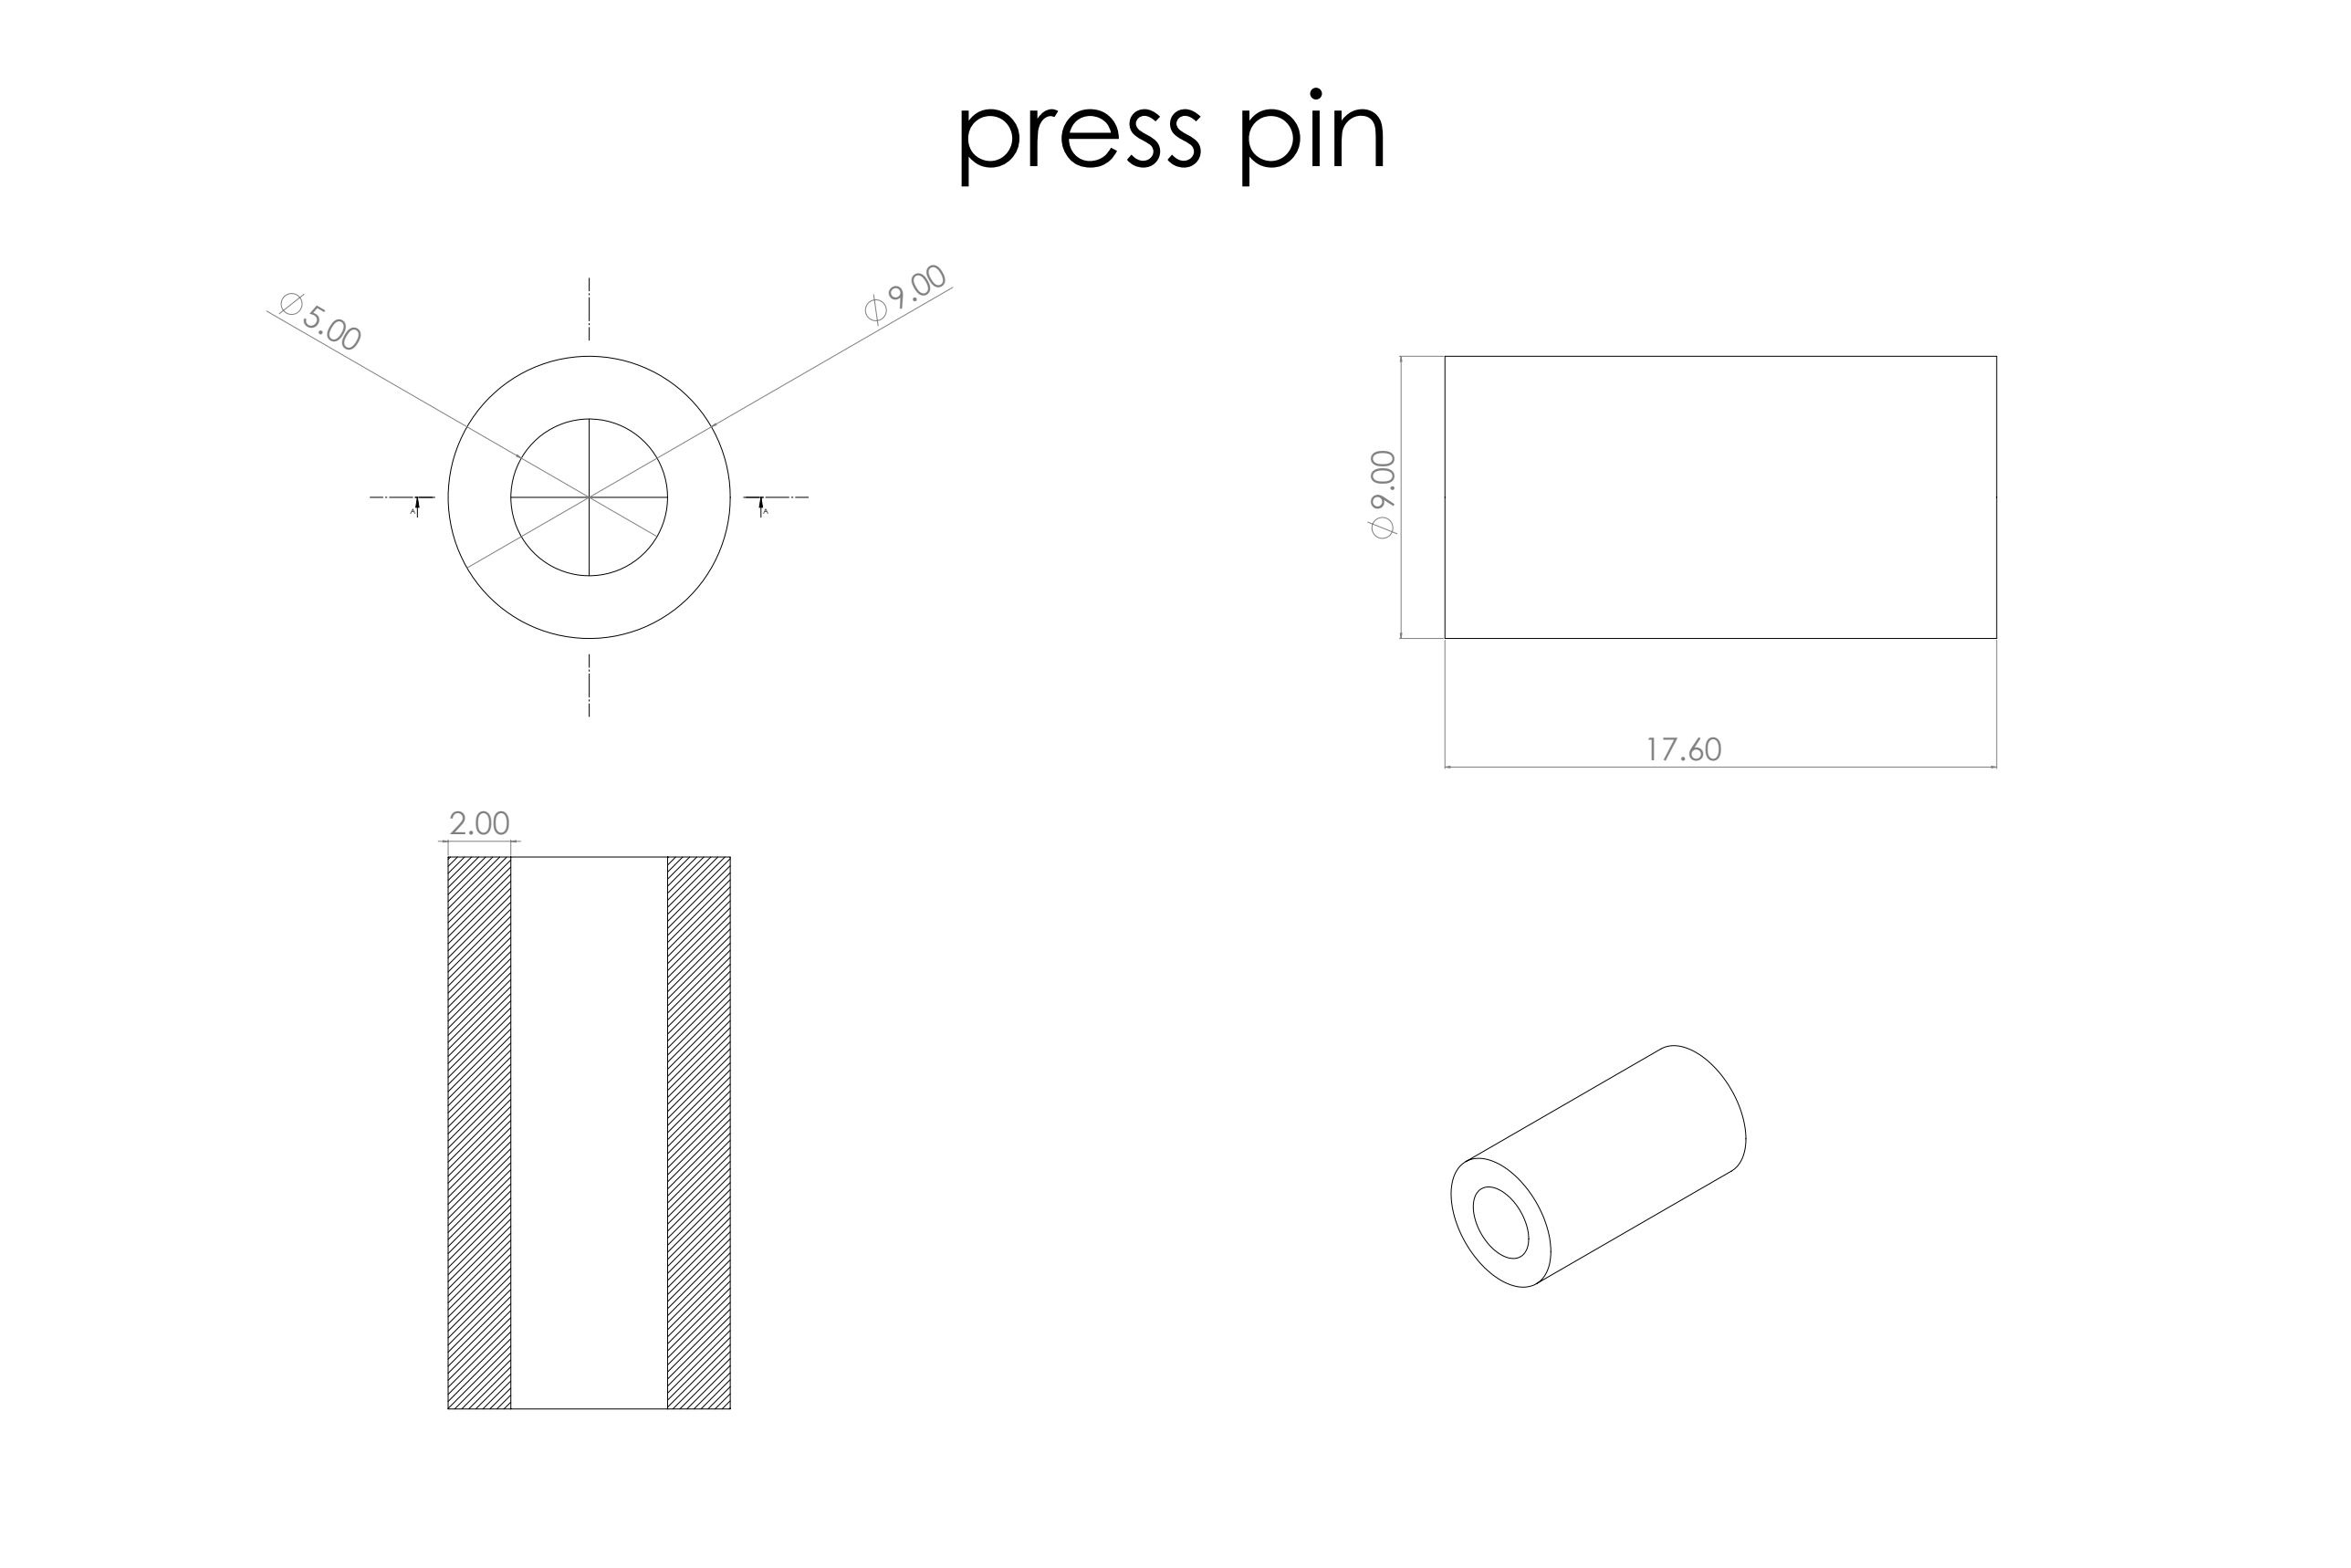
ISO-10303-21;
HEADER;
FILE_DESCRIPTION (('STEP AP214'),
    '1' );
FILE_NAME ('Press Pin.step',
    '2026-10-24T22:54:28',
    ( '' ),
    ( '' ),
    'SwSTEP 2.0',
    'SolidWorks 2025',
    '' );
FILE_SCHEMA (( 'AUTOMOTIVE_DESIGN' ));
ENDSEC;

DATA;
#29=ORIENTED_EDGE ( 'NONE', *, *, #33251, .T. ) ;
#151=( NAMED_UNIT ( * ) PLANE_ANGLE_UNIT ( ) SI_UNIT ( $, .RADIAN. ) );
#350=CARTESIAN_POINT ( 'NONE',  ( -72.95330471031414277, 33.71485196875532608, 8.800414904976364028 ) ) ;
#530=VERTEX_POINT ( 'NONE', #38113 ) ;
#618=DIRECTION ( 'NONE',  ( -0.000000000000000000, -0.000000000000000000, -1.000000000000000000 ) ) ;
#809=ADVANCED_FACE ( 'NONE', ( #1232 ), #9869, .F. ) ;
#1232=FACE_OUTER_BOUND ( 'NONE', #23037, .T. ) ;
#1366=SHAPE_DEFINITION_REPRESENTATION ( #33255, #27999 ) ;
#1487=CARTESIAN_POINT ( 'NONE',  ( -70.95330471031414277, 33.71485196875532608, 8.800414904976364028 ) ) ;
#2187=CARTESIAN_POINT ( 'NONE',  ( -77.95330471031414277, 33.71485196875532608, 21.52833696633422988 ) ) ;
#2281=DIRECTION ( 'NONE',  ( 0.000000000000000000, 0.000000000000000000, 1.000000000000000000 ) ) ;
#2378=VERTEX_POINT ( 'NONE', #25159 ) ;
#2401=LINE ( 'NONE', #2187, #2524 ) ;
#2415=DIRECTION ( 'NONE',  ( 1.000000000000000000, 0.000000000000000000, 0.000000000000000000 ) ) ;
#2524=VECTOR ( 'NONE', #17586, 1000.000000000000000 ) ;
#2592=CARTESIAN_POINT ( 'NONE',  ( -75.45330471031414277, 33.71485196875532608, 8.800414904976364028 ) ) ;
#2681=ORIENTED_EDGE ( 'NONE', *, *, #18740, .T. ) ;
#2880=STYLED_ITEM('',(#40759),#26229);
#2983=CARTESIAN_POINT ( 'NONE',  ( -77.95330471031414277, 33.71485196875532608, -8.800414904976364028 ) ) ;
#3239=DIRECTION ( 'NONE',  ( 1.000000000000000000, 0.000000000000000000, 0.000000000000000000 ) ) ;
#3272=FACE_OUTER_BOUND ( 'NONE', #21935, .T. ) ;
#3553=DIRECTION ( 'NONE',  ( 1.000000000000000000, 0.000000000000000000, 0.000000000000000000 ) ) ;
#3611=AXIS2_PLACEMENT_3D ( 'NONE', #8446, #26995, #5378 ) ;
#3661=ORIENTED_EDGE ( 'NONE', *, *, #24979, .F. ) ;
#3684=DIRECTION ( 'NONE',  ( -0.000000000000000000, 0.000000000000000000, 1.000000000000000000 ) ) ;
#4380=ADVANCED_BREP_SHAPE_REPRESENTATION ( '', ( #26229, #30744 ), #8364 ) ;
#4541=VERTEX_POINT ( 'NONE', #1487 ) ;
#4809=VERTEX_POINT ( 'NONE', #25758 ) ;
#4902=DIRECTION ( 'NONE',  ( 1.000000000000000000, 0.000000000000000000, -0.000000000000000000 ) ) ;
#5038=EDGE_CURVE ( 'NONE', #4541, #2378, #8198, .T. ) ;
#5067=CARTESIAN_POINT ( 'NONE',  ( -75.45330471031414277, 33.71485196875532608, 21.52833696633422988 ) ) ;
#5378=DIRECTION ( 'NONE',  ( 1.000000000000000000, 0.000000000000000000, 0.000000000000000000 ) ) ;
#5502=AXIS2_PLACEMENT_3D ( 'NONE', #32883, #20106, #23207 ) ;
#5704=UNCERTAINTY_MEASURE_WITH_UNIT (LENGTH_MEASURE( 1.000000000000000082E-05 ), #38397, 'distance_accuracy_value', 'NONE');
#6398=EDGE_CURVE ( 'NONE', #530, #35439, #2401, .T. ) ;
#6470=AXIS2_PLACEMENT_3D ( 'NONE', #8776, #37197, #24860 ) ;
#6752=PLANE ( 'NONE',  #38681 ) ;
#6765=ORIENTED_EDGE ( 'NONE', *, *, #30608, .T. ) ;
#6800=MECHANICAL_DESIGN_GEOMETRIC_PRESENTATION_REPRESENTATION('',(#2880),#15985);
#6851=AXIS2_PLACEMENT_3D ( 'NONE', #19276, #16183, #15784 ) ;
#7085=ADVANCED_FACE ( 'NONE', ( #33735, #14556 ), #27541, .F. ) ;
#7104=DIRECTION ( 'NONE',  ( -0.000000000000000000, -0.000000000000000000, -1.000000000000000000 ) ) ;
#7678=CIRCLE ( 'NONE', #12943, 4.500000000000003553 ) ;
#8198=LINE ( 'NONE', #17669, #16532 ) ;
#8364=( GEOMETRIC_REPRESENTATION_CONTEXT ( 3 ) GLOBAL_UNCERTAINTY_ASSIGNED_CONTEXT ( ( #5704 ) ) GLOBAL_UNIT_ASSIGNED_CONTEXT ( ( #38397, #151, #28335 ) ) REPRESENTATION_CONTEXT ( 'NONE', 'WORKASPACE' ) );
#8438=PRODUCT_DEFINITION ( 'UNKNOWN', '', #13007, #18868 ) ;
#8446=CARTESIAN_POINT ( 'NONE',  ( -75.45330471031414277, 33.71485196875532608, 8.800414904976364028 ) ) ;
#8776=CARTESIAN_POINT ( 'NONE',  ( -75.45330471031414277, 33.71485196875532608, 21.52833696633422988 ) ) ;
#8933=AXIS2_PLACEMENT_3D ( 'NONE', #5067, #29975, #35965 ) ;
#8934=CIRCLE ( 'NONE', #28011, 4.500000000000003553 ) ;
#9175=ORIENTED_EDGE ( 'NONE', *, *, #6398, .T. ) ;
#9445=ORIENTED_EDGE ( 'NONE', *, *, #22485, .T. ) ;
#9485=DIRECTION ( 'NONE',  ( 0.000000000000000000, 0.000000000000000000, 1.000000000000000000 ) ) ;
#9531=AXIS2_PLACEMENT_3D ( 'NONE', #14115, #35964, #35575 ) ;
#9831=FACE_BOUND ( 'NONE', #16930, .T. ) ;
#9869=CYLINDRICAL_SURFACE ( 'NONE', #32843, 2.500000000000002220 ) ;
#11002=ADVANCED_FACE ( 'NONE', ( #9831, #34977 ), #6752, .T. ) ;
#11346=VERTEX_POINT ( 'NONE', #31824 ) ;
#11702=AXIS2_PLACEMENT_3D ( 'NONE', #14762, #30432, #4902 ) ;
#11915=CARTESIAN_POINT ( 'NONE',  ( -75.45330471031414277, 33.71485196875532608, -8.800414904976364028 ) ) ;
#12435=DIRECTION ( 'NONE',  ( -0.000000000000000000, 0.000000000000000000, 1.000000000000000000 ) ) ;
#12589=ORIENTED_EDGE ( 'NONE', *, *, #19173, .T. ) ;
#12695=EDGE_LOOP ( 'NONE', ( #14818, #9445, #9175, #30546 ) ) ;
#12943=AXIS2_PLACEMENT_3D ( 'NONE', #37766, #40440, #3239 ) ;
#13007=PRODUCT_DEFINITION_FORMATION_WITH_SPECIFIED_SOURCE ( 'ANY', '', #15521, .NOT_KNOWN. ) ;
#14115=CARTESIAN_POINT ( 'NONE',  ( -75.45330471031414277, 33.71485196875532608, 21.52833696633422988 ) ) ;
#14483=ORIENTED_EDGE ( 'NONE', *, *, #17982, .F. ) ;
#14500=ADVANCED_FACE ( 'NONE', ( #39021 ), #33286, .T. ) ;
#14556=FACE_BOUND ( 'NONE', #34340, .T. ) ;
#14762=CARTESIAN_POINT ( 'NONE',  ( -75.45330471031414277, 33.71485196875532608, -8.800414904976364028 ) ) ;
#14800=( LENGTH_UNIT ( ) NAMED_UNIT ( * ) SI_UNIT ( .MILLI., .METRE. ) );
#14806=DIRECTION ( 'NONE',  ( 1.000000000000000000, 0.000000000000000000, 0.000000000000000000 ) ) ;
#14818=ORIENTED_EDGE ( 'NONE', *, *, #35359, .F. ) ;
#15469=VECTOR ( 'NONE', #26062, 1000.000000000000000 ) ;
#15521=PRODUCT ( 'Press Pin', 'Press Pin', '', ( #29549 ) ) ;
#15616=EDGE_CURVE ( 'NONE', #27554, #35439, #29833, .T. ) ;
#15784=DIRECTION ( 'NONE',  ( 1.000000000000000000, 0.000000000000000000, 0.000000000000000000 ) ) ;
#15979=UNCERTAINTY_MEASURE_WITH_UNIT (LENGTH_MEASURE( 1.000000000000000082E-05 ), #14800, 'distance_accuracy_value', 'NONE');
#15985=( GEOMETRIC_REPRESENTATION_CONTEXT ( 3 ) GLOBAL_UNCERTAINTY_ASSIGNED_CONTEXT ( ( #15979 ) ) GLOBAL_UNIT_ASSIGNED_CONTEXT ( ( #14800, #35844, #16837 ) ) REPRESENTATION_CONTEXT ( 'NONE', 'WORKASPACE' ) );
#15989=CYLINDRICAL_SURFACE ( 'NONE', #6470, 4.500000000000003553 ) ;
#16183=DIRECTION ( 'NONE',  ( 0.000000000000000000, 0.000000000000000000, 1.000000000000000000 ) ) ;
#16208=DIRECTION ( 'NONE',  ( 1.000000000000000000, 0.000000000000000000, 0.000000000000000000 ) ) ;
#16245=CARTESIAN_POINT ( 'NONE',  ( -75.45330471031414277, 33.71485196875532608, 21.52833696633422988 ) ) ;
#16532=VECTOR ( 'NONE', #39707, 1000.000000000000000 ) ;
#16837=( NAMED_UNIT ( * ) SI_UNIT ( $, .STERADIAN. ) SOLID_ANGLE_UNIT ( ) );
#16930=EDGE_LOOP ( 'NONE', ( #32550, #37840 ) ) ;
#17023=ORIENTED_EDGE ( 'NONE', *, *, #19173, .F. ) ;
#17586=DIRECTION ( 'NONE',  ( -0.000000000000000000, -0.000000000000000000, -1.000000000000000000 ) ) ;
#17669=CARTESIAN_POINT ( 'NONE',  ( -70.95330471031414277, 33.71485196875532608, 21.52833696633422988 ) ) ;
#17982=EDGE_CURVE ( 'NONE', #4809, #4541, #33262, .T. ) ;
#18055=ORIENTED_EDGE ( 'NONE', *, *, #30608, .F. ) ;
#18740=EDGE_CURVE ( 'NONE', #2378, #11346, #8934, .T. ) ;
#18868=PRODUCT_DEFINITION_CONTEXT ( 'detailed design', #27896, 'design' ) ;
#19173=EDGE_CURVE ( 'NONE', #4809, #11346, #35335, .T. ) ;
#19276=CARTESIAN_POINT ( 'NONE',  ( -75.45330471031414277, 33.71485196875532608, -8.800414904976364028 ) ) ;
#19972=DIRECTION ( 'NONE',  ( -0.000000000000000000, 0.000000000000000000, 1.000000000000000000 ) ) ;
#20065=CARTESIAN_POINT ( 'NONE',  ( -79.95330471031414277, 33.71485196875532608, 21.52833696633422988 ) ) ;
#20103=AXIS2_PLACEMENT_3D ( 'NONE', #2592, #12435, #40029 ) ;
#20106=DIRECTION ( 'NONE',  ( 0.000000000000000000, 0.000000000000000000, 1.000000000000000000 ) ) ;
#20567=CARTESIAN_POINT ( 'NONE',  ( -75.45330471031414277, 33.71485196875532608, 8.800414904976364028 ) ) ;
#20960=ORIENTED_EDGE ( 'NONE', *, *, #18740, .F. ) ;
#21073=ADVANCED_FACE ( 'NONE', ( #39637 ), #29769, .F. ) ;
#21335=CIRCLE ( 'NONE', #3611, 2.500000000000002220 ) ;
#21847=EDGE_CURVE ( 'NONE', #530, #24953, #21335, .T. ) ;
#21935=EDGE_LOOP ( 'NONE', ( #18055, #23977, #2681, #17023 ) ) ;
#22485=EDGE_CURVE ( 'NONE', #24953, #530, #31248, .T. ) ;
#22634=CIRCLE ( 'NONE', #29203, 2.500000000000002220 ) ;
#22658=ORIENTED_EDGE ( 'NONE', *, *, #24979, .T. ) ;
#23037=EDGE_LOOP ( 'NONE', ( #36726, #36527, #32521, #33328 ) ) ;
#23207=DIRECTION ( 'NONE',  ( 1.000000000000000000, 0.000000000000000000, 0.000000000000000000 ) ) ;
#23855=DIRECTION ( 'NONE',  ( 1.000000000000000000, 0.000000000000000000, 0.000000000000000000 ) ) ;
#23977=ORIENTED_EDGE ( 'NONE', *, *, #5038, .T. ) ;
#24592=CIRCLE ( 'NONE', #6851, 4.500000000000003553 ) ;
#24860=DIRECTION ( 'NONE',  ( -1.000000000000000000, 0.000000000000000000, 0.000000000000000000 ) ) ;
#24953=VERTEX_POINT ( 'NONE', #350 ) ;
#24979=EDGE_CURVE ( 'NONE', #11346, #2378, #24592, .T. ) ;
#25159=CARTESIAN_POINT ( 'NONE',  ( -70.95330471031414277, 33.71485196875532608, -8.800414904976364028 ) ) ;
#25758=CARTESIAN_POINT ( 'NONE',  ( -79.95330471031414277, 33.71485196875532608, 8.800414904976364028 ) ) ;
#26062=DIRECTION ( 'NONE',  ( -0.000000000000000000, -0.000000000000000000, -1.000000000000000000 ) ) ;
#26229=MANIFOLD_SOLID_BREP ( 'Boss-Extrude7', #34124 ) ;
#26585=APPLICATION_CONTEXT ( 'automotive_design' ) ;
#26995=DIRECTION ( 'NONE',  ( -0.000000000000000000, 0.000000000000000000, 1.000000000000000000 ) ) ;
#27266=ORIENTED_EDGE ( 'NONE', *, *, #5038, .F. ) ;
#27541=PLANE ( 'NONE',  #11702 ) ;
#27554=VERTEX_POINT ( 'NONE', #32887 ) ;
#27896=APPLICATION_CONTEXT ( 'automotive_design' ) ;
#27999=SHAPE_REPRESENTATION ( 'Press Pin', ( #30744 ), #8364 ) ;
#28011=AXIS2_PLACEMENT_3D ( 'NONE', #30606, #33501, #2415 ) ;
#28335=( NAMED_UNIT ( * ) SI_UNIT ( $, .STERADIAN. ) SOLID_ANGLE_UNIT ( ) );
#28539=SHAPE_REPRESENTATION_RELATIONSHIP ( 'NONE' , 'NONE' ,  #27999, #4380 ) ;
#29147=CARTESIAN_POINT ( 'NONE',  ( -72.95330471031414277, 33.71485196875532608, 21.52833696633422988 ) ) ;
#29203=AXIS2_PLACEMENT_3D ( 'NONE', #11915, #2281, #14806 ) ;
#29549=PRODUCT_CONTEXT ( 'NONE', #26585, 'mechanical' ) ;
#29769=CYLINDRICAL_SURFACE ( 'NONE', #9531, 2.500000000000002220 ) ;
#29833=CIRCLE ( 'NONE', #5502, 2.500000000000002220 ) ;
#29975=DIRECTION ( 'NONE',  ( -0.000000000000000000, -0.000000000000000000, -1.000000000000000000 ) ) ;
#29993=ADVANCED_FACE ( 'NONE', ( #3272 ), #15989, .T. ) ;
#30432=DIRECTION ( 'NONE',  ( 0.000000000000000000, 0.000000000000000000, 1.000000000000000000 ) ) ;
#30546=ORIENTED_EDGE ( 'NONE', *, *, #15616, .F. ) ;
#30591=VECTOR ( 'NONE', #7104, 1000.000000000000000 ) ;
#30606=CARTESIAN_POINT ( 'NONE',  ( -75.45330471031414277, 33.71485196875532608, -8.800414904976364028 ) ) ;
#30608=EDGE_CURVE ( 'NONE', #4541, #4809, #7678, .T. ) ;
#30744=AXIS2_PLACEMENT_3D ( 'NONE', #35448, #9485, #3553 ) ;
#31248=CIRCLE ( 'NONE', #36490, 2.500000000000002220 ) ;
#31824=CARTESIAN_POINT ( 'NONE',  ( -79.95330471031414277, 33.71485196875532608, -8.800414904976364028 ) ) ;
#31873=CARTESIAN_POINT ( 'NONE',  ( -94.24726447194083789, -65.19654454972992141, 8.800414904976364028 ) ) ;
#32521=ORIENTED_EDGE ( 'NONE', *, *, #33251, .F. ) ;
#32550=ORIENTED_EDGE ( 'NONE', *, *, #21847, .F. ) ;
#32843=AXIS2_PLACEMENT_3D ( 'NONE', #16245, #618, #38264 ) ;
#32883=CARTESIAN_POINT ( 'NONE',  ( -75.45330471031414277, 33.71485196875532608, -8.800414904976364028 ) ) ;
#32887=CARTESIAN_POINT ( 'NONE',  ( -72.95330471031414277, 33.71485196875532608, -8.800414904976364028 ) ) ;
#33251=EDGE_CURVE ( 'NONE', #35439, #27554, #22634, .T. ) ;
#33255=PRODUCT_DEFINITION_SHAPE ( 'NONE', 'NONE',  #8438 ) ;
#33262=CIRCLE ( 'NONE', #20103, 4.500000000000003553 ) ;
#33286=CYLINDRICAL_SURFACE ( 'NONE', #8933, 4.500000000000003553 ) ;
#33328=ORIENTED_EDGE ( 'NONE', *, *, #6398, .F. ) ;
#33501=DIRECTION ( 'NONE',  ( 0.000000000000000000, 0.000000000000000000, 1.000000000000000000 ) ) ;
#33735=FACE_OUTER_BOUND ( 'NONE', #35066, .T. ) ;
#34124=CLOSED_SHELL ( 'NONE', ( #809, #29993, #14500, #7085, #21073, #11002 ) ) ;
#34340=EDGE_LOOP ( 'NONE', ( #29, #37157 ) ) ;
#34977=FACE_OUTER_BOUND ( 'NONE', #35239, .T. ) ;
#35066=EDGE_LOOP ( 'NONE', ( #3661, #20960 ) ) ;
#35239=EDGE_LOOP ( 'NONE', ( #39195, #6765 ) ) ;
#35335=LINE ( 'NONE', #20065, #30591 ) ;
#35359=EDGE_CURVE ( 'NONE', #24953, #27554, #38391, .T. ) ;
#35439=VERTEX_POINT ( 'NONE', #2983 ) ;
#35448=CARTESIAN_POINT ( 'NONE',  ( 0.000000000000000000, 0.000000000000000000, 0.000000000000000000 ) ) ;
#35575=DIRECTION ( 'NONE',  ( -1.000000000000000000, 0.000000000000000000, 0.000000000000000000 ) ) ;
#35844=( NAMED_UNIT ( * ) PLANE_ANGLE_UNIT ( ) SI_UNIT ( $, .RADIAN. ) );
#35964=DIRECTION ( 'NONE',  ( -0.000000000000000000, -0.000000000000000000, -1.000000000000000000 ) ) ;
#35965=DIRECTION ( 'NONE',  ( -1.000000000000000000, 0.000000000000000000, 0.000000000000000000 ) ) ;
#36490=AXIS2_PLACEMENT_3D ( 'NONE', #20567, #19972, #23855 ) ;
#36527=ORIENTED_EDGE ( 'NONE', *, *, #35359, .T. ) ;
#36726=ORIENTED_EDGE ( 'NONE', *, *, #21847, .T. ) ;
#37157=ORIENTED_EDGE ( 'NONE', *, *, #15616, .T. ) ;
#37197=DIRECTION ( 'NONE',  ( -0.000000000000000000, -0.000000000000000000, -1.000000000000000000 ) ) ;
#37766=CARTESIAN_POINT ( 'NONE',  ( -75.45330471031414277, 33.71485196875532608, 8.800414904976364028 ) ) ;
#37840=ORIENTED_EDGE ( 'NONE', *, *, #22485, .F. ) ;
#38113=CARTESIAN_POINT ( 'NONE',  ( -77.95330471031414277, 33.71485196875532608, 8.800414904976364028 ) ) ;
#38264=DIRECTION ( 'NONE',  ( -1.000000000000000000, 0.000000000000000000, 0.000000000000000000 ) ) ;
#38391=LINE ( 'NONE', #29147, #15469 ) ;
#38397=( LENGTH_UNIT ( ) NAMED_UNIT ( * ) SI_UNIT ( .MILLI., .METRE. ) );
#38681=AXIS2_PLACEMENT_3D ( 'NONE', #31873, #3684, #16208 ) ;
#39021=FACE_OUTER_BOUND ( 'NONE', #39092, .T. ) ;
#39092=EDGE_LOOP ( 'NONE', ( #27266, #14483, #12589, #22658 ) ) ;
#39195=ORIENTED_EDGE ( 'NONE', *, *, #17982, .T. ) ;
#39637=FACE_OUTER_BOUND ( 'NONE', #12695, .T. ) ;
#39707=DIRECTION ( 'NONE',  ( -0.000000000000000000, -0.000000000000000000, -1.000000000000000000 ) ) ;
#40029=DIRECTION ( 'NONE',  ( 1.000000000000000000, 0.000000000000000000, 0.000000000000000000 ) ) ;
#40440=DIRECTION ( 'NONE',  ( -0.000000000000000000, 0.000000000000000000, 1.000000000000000000 ) ) ;
#40753=COLOUR_RGB('Grey',0.48,0.52,0.57);
#40754=FILL_AREA_STYLE_COLOUR('',#40753);
#40755=FILL_AREA_STYLE('',(#40754));
#40756=SURFACE_STYLE_FILL_AREA(#40755);
#40757=SURFACE_SIDE_STYLE('',(#40756));
#40758=SURFACE_STYLE_USAGE(.BOTH.,#40757);
#40759=PRESENTATION_STYLE_ASSIGNMENT((#40758));
ENDSEC;
END-ISO-10303-21;
